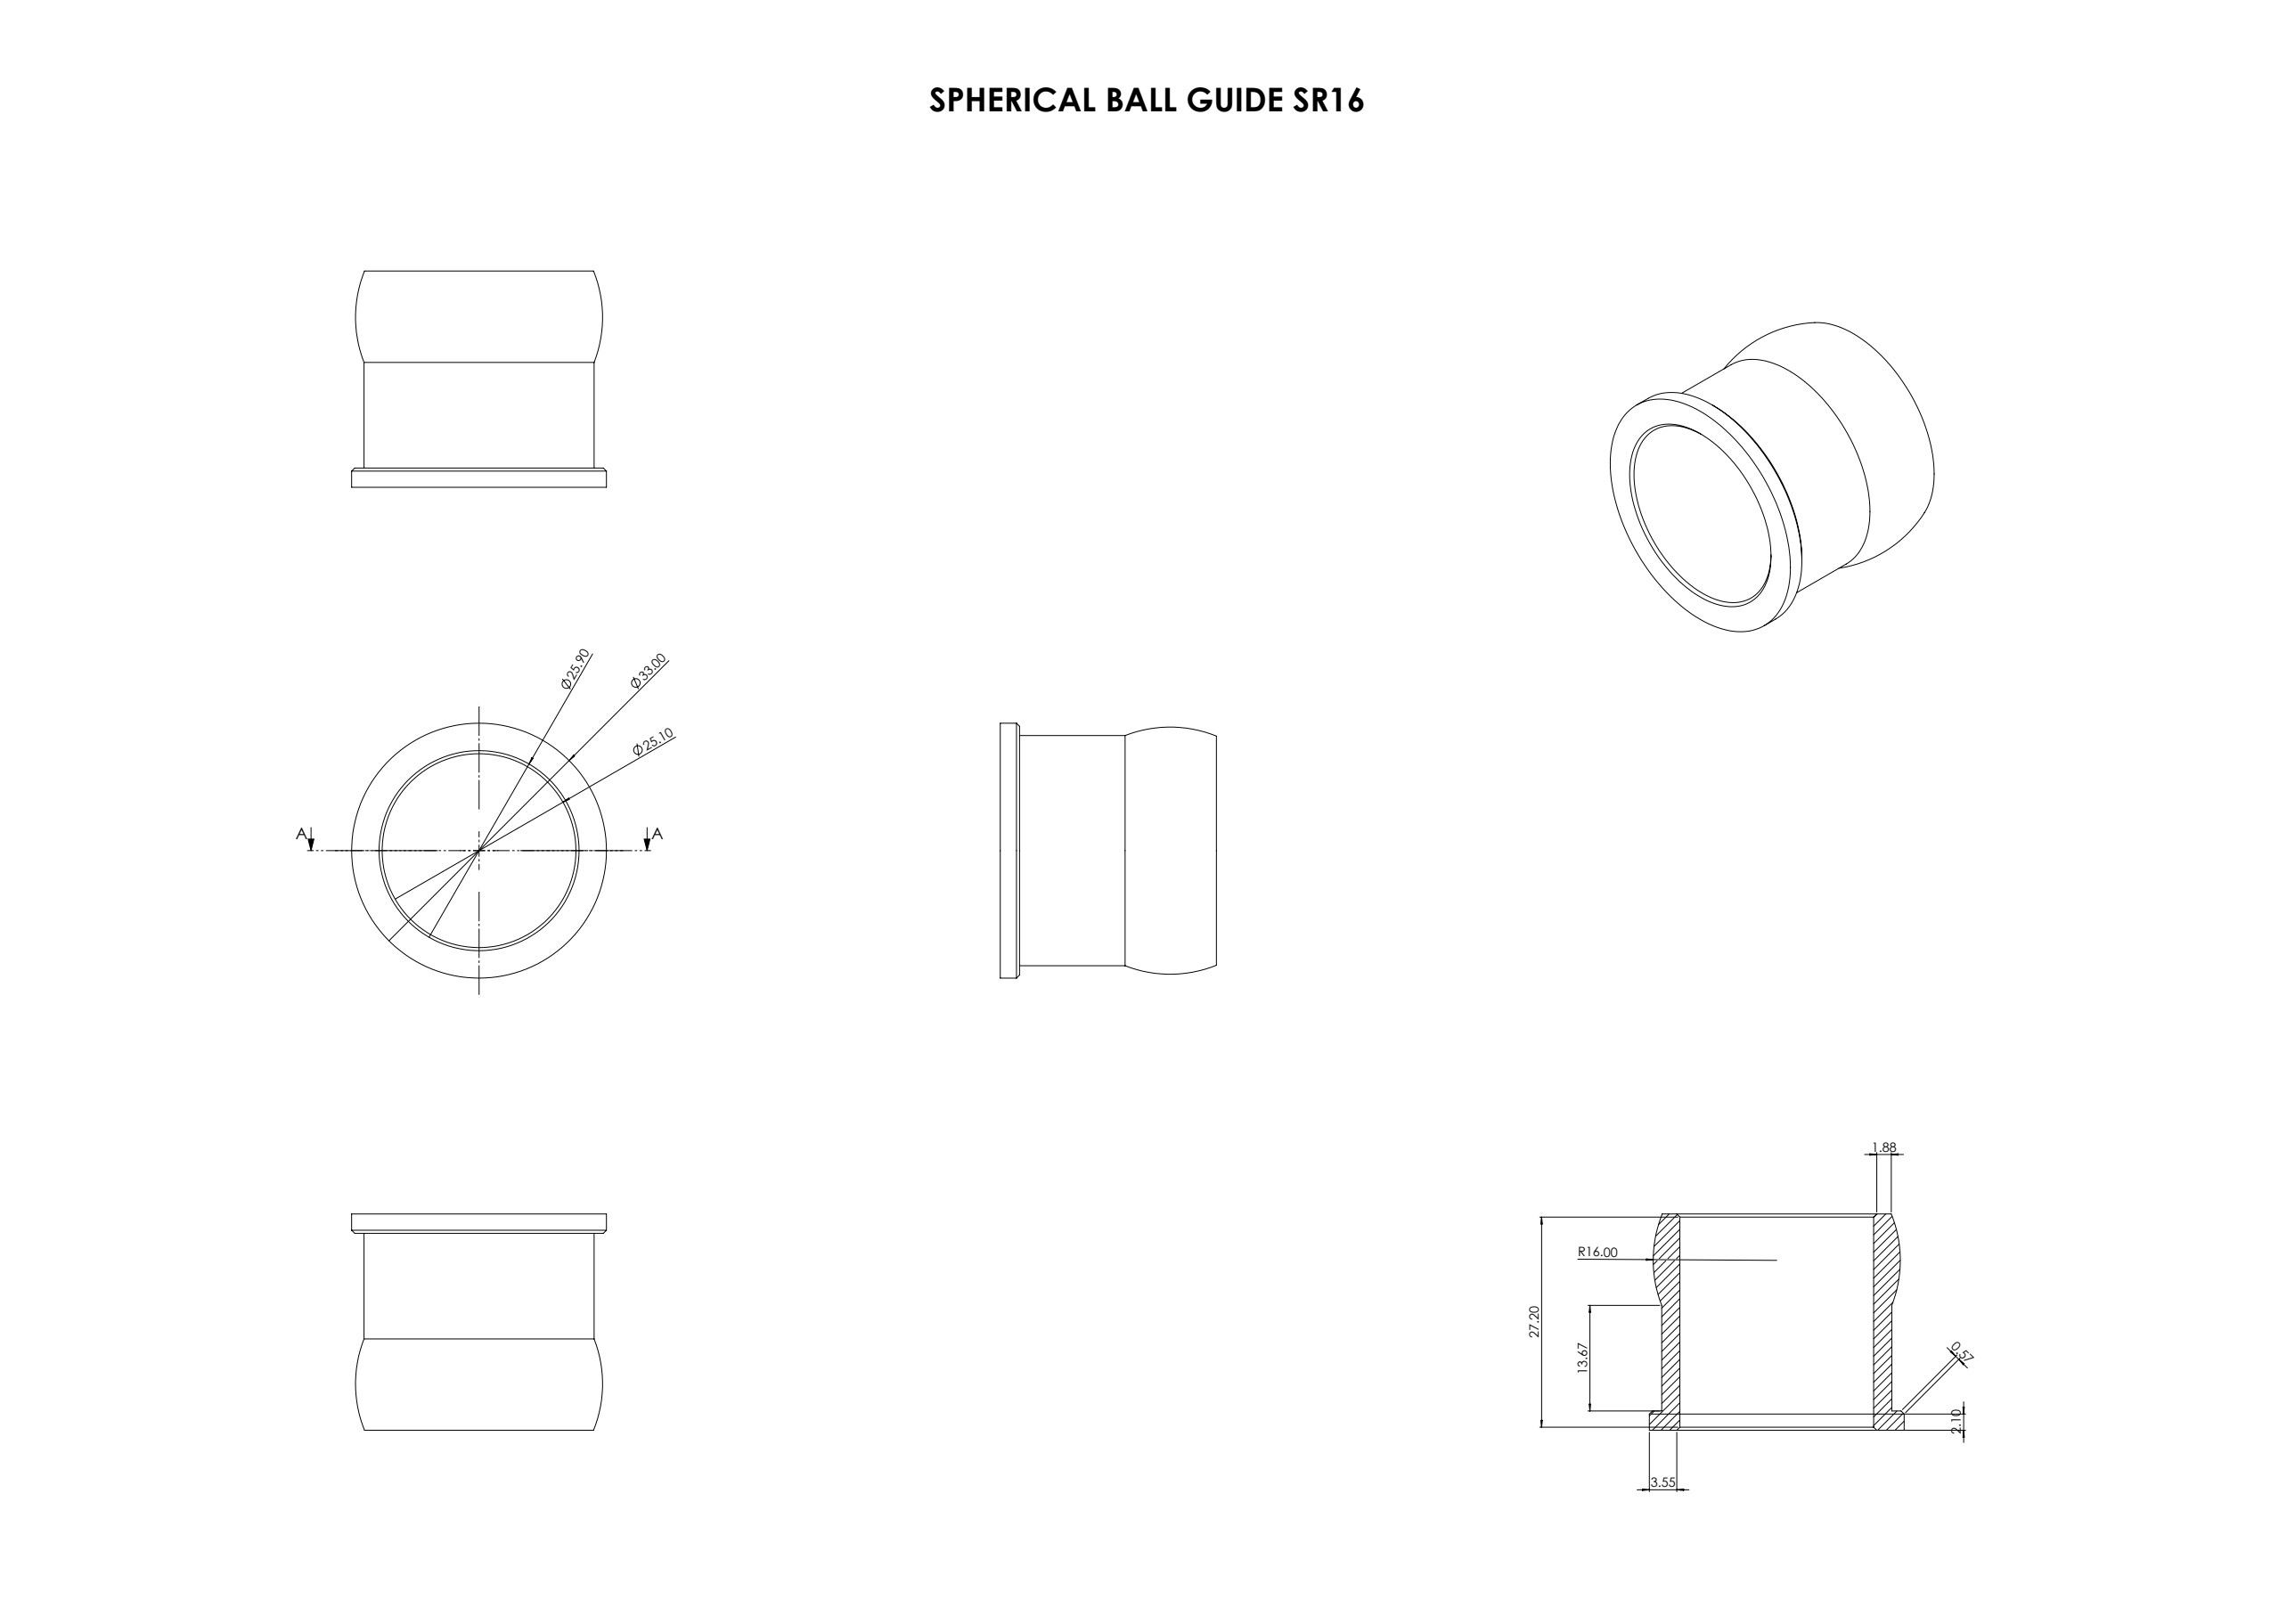
ISO-10303-21;
HEADER;
/* Generated by software containing ST-Developer
 * from STEP Tools, Inc. (www.steptools.com) 
 */

FILE_DESCRIPTION(
/* description */ (''),
/* implementation_level */ '2;1');

FILE_NAME(
/* name */ '09_Spherical_Ball_Guide_SR16.step',
/* time_stamp */ '2026-10-23T00:52:27+05:00',
/* author */ (''),
/* organization */ (''),
/* preprocessor_version */ 'ST-DEVELOPER v20.2',
/* originating_system */ 'Autodesk Translation Framework v15.15.0.0',
/* authorisation */ '');

FILE_SCHEMA (('AUTOMOTIVE_DESIGN { 1 0 10303 214 3 1 1 }'));
ENDSEC;

DATA;
#10=MECHANICAL_DESIGN_GEOMETRIC_PRESENTATION_REPRESENTATION('',(#1549),#59204);
#1509=SHAPE_REPRESENTATION_RELATIONSHIP('SRR','None',#59298,#1529);
#1529=ADVANCED_BREP_SHAPE_REPRESENTATION('',(#1576),#59185);
#1549=STYLED_ITEM('',(#59600),#1576);
#1576=MANIFOLD_SOLID_BREP('Ball guide',#22805);
#1596=SPHERICAL_SURFACE('',#23143,1.6);
#1619=FACE_BOUND('',#4029,.T.);
#1620=FACE_BOUND('',#4033,.T.);
#1621=FACE_BOUND('',#4038,.T.);
#1812=PLANE('',#23127);
#1813=PLANE('',#23133);
#1814=PLANE('',#23141);
#2419=CYLINDRICAL_SURFACE('',#23124,1.49);
#2420=CYLINDRICAL_SURFACE('',#23131,1.65);
#2421=CYLINDRICAL_SURFACE('',#23137,1.255);
#2702=FACE_OUTER_BOUND('',#4027,.T.);
#2703=FACE_OUTER_BOUND('',#4028,.T.);
#2704=FACE_OUTER_BOUND('',#4030,.T.);
#2705=FACE_OUTER_BOUND('',#4031,.T.);
#2706=FACE_OUTER_BOUND('',#4032,.T.);
#2707=FACE_OUTER_BOUND('',#4034,.T.);
#2708=FACE_OUTER_BOUND('',#4035,.T.);
#2709=FACE_OUTER_BOUND('',#4036,.T.);
#2710=FACE_OUTER_BOUND('',#4037,.T.);
#2711=FACE_OUTER_BOUND('',#4039,.T.);
#4027=EDGE_LOOP('',(#14808,#14809,#14810,#14811));
#4028=EDGE_LOOP('',(#14812));
#4029=EDGE_LOOP('',(#14813));
#4030=EDGE_LOOP('',(#14814,#14815,#14816,#14817));
#4031=EDGE_LOOP('',(#14818,#14819,#14820,#14821));
#4032=EDGE_LOOP('',(#14822));
#4033=EDGE_LOOP('',(#14823));
#4034=EDGE_LOOP('',(#14824,#14825,#14826,#14827));
#4035=EDGE_LOOP('',(#14828,#14829,#14830,#14831));
#4036=EDGE_LOOP('',(#14832,#14833,#14834,#14835));
#4037=EDGE_LOOP('',(#14836));
#4038=EDGE_LOOP('',(#14837));
#4039=EDGE_LOOP('',(#14838,#14839,#14840,#14841));
#5520=LINE('',#30846,#6953);
#5521=LINE('',#30854,#6954);
#5522=LINE('',#30858,#6955);
#5523=LINE('',#30864,#6956);
#5524=LINE('',#30868,#6957);
#5525=LINE('',#30872,#6958);
#6953=VECTOR('',#25308,1.49);
#6954=VECTOR('',#25319,1.63);
#6955=VECTOR('',#25324,1.65);
#6956=VECTOR('',#25331,1.275);
#6957=VECTOR('',#25336,1.255);
#6958=VECTOR('',#25341,1.275);
#8399=CIRCLE('',#23125,1.49);
#8400=CIRCLE('',#23126,1.49);
#8401=CIRCLE('',#23128,1.61);
#8402=CIRCLE('',#23130,1.65);
#8403=CIRCLE('',#23132,1.65);
#8404=CIRCLE('',#23134,1.295);
#8405=CIRCLE('',#23136,1.255);
#8406=CIRCLE('',#23138,1.255);
#8407=CIRCLE('',#23140,1.295);
#8408=CIRCLE('',#23142,1.48323969741913);
#8409=CIRCLE('',#23144,1.6);
#9234=VERTEX_POINT('',#30843);
#9235=VERTEX_POINT('',#30845);
#9236=VERTEX_POINT('',#30849);
#9237=VERTEX_POINT('',#30852);
#9238=VERTEX_POINT('',#30856);
#9239=VERTEX_POINT('',#30860);
#9240=VERTEX_POINT('',#30863);
#9241=VERTEX_POINT('',#30867);
#9242=VERTEX_POINT('',#30871);
#9243=VERTEX_POINT('',#30875);
#11408=EDGE_CURVE('',#9234,#9234,#8399,.T.);
#11409=EDGE_CURVE('',#9234,#9235,#5520,.T.);
#11410=EDGE_CURVE('',#9235,#9235,#8400,.T.);
#11411=EDGE_CURVE('',#9236,#9236,#8401,.T.);
#11412=EDGE_CURVE('',#9237,#9237,#8402,.T.);
#11413=EDGE_CURVE('',#9237,#9236,#5521,.T.);
#11414=EDGE_CURVE('',#9238,#9238,#8403,.T.);
#11415=EDGE_CURVE('',#9238,#9237,#5522,.T.);
#11416=EDGE_CURVE('',#9239,#9239,#8404,.T.);
#11417=EDGE_CURVE('',#9239,#9240,#5523,.T.);
#11418=EDGE_CURVE('',#9240,#9240,#8405,.T.);
#11419=EDGE_CURVE('',#9240,#9241,#5524,.T.);
#11420=EDGE_CURVE('',#9241,#9241,#8406,.T.);
#11421=EDGE_CURVE('',#9241,#9242,#5525,.T.);
#11422=EDGE_CURVE('',#9242,#9242,#8407,.T.);
#11423=EDGE_CURVE('',#9243,#9243,#8408,.T.);
#11424=EDGE_CURVE('',#9235,#9243,#8409,.T.);
#14808=ORIENTED_EDGE('',*,*,#11408,.F.);
#14809=ORIENTED_EDGE('',*,*,#11409,.T.);
#14810=ORIENTED_EDGE('',*,*,#11410,.T.);
#14811=ORIENTED_EDGE('',*,*,#11409,.F.);
#14812=ORIENTED_EDGE('',*,*,#11411,.F.);
#14813=ORIENTED_EDGE('',*,*,#11408,.T.);
#14814=ORIENTED_EDGE('',*,*,#11412,.F.);
#14815=ORIENTED_EDGE('',*,*,#11413,.T.);
#14816=ORIENTED_EDGE('',*,*,#11411,.T.);
#14817=ORIENTED_EDGE('',*,*,#11413,.F.);
#14818=ORIENTED_EDGE('',*,*,#11414,.F.);
#14819=ORIENTED_EDGE('',*,*,#11415,.T.);
#14820=ORIENTED_EDGE('',*,*,#11412,.T.);
#14821=ORIENTED_EDGE('',*,*,#11415,.F.);
#14822=ORIENTED_EDGE('',*,*,#11414,.T.);
#14823=ORIENTED_EDGE('',*,*,#11416,.F.);
#14824=ORIENTED_EDGE('',*,*,#11416,.T.);
#14825=ORIENTED_EDGE('',*,*,#11417,.T.);
#14826=ORIENTED_EDGE('',*,*,#11418,.F.);
#14827=ORIENTED_EDGE('',*,*,#11417,.F.);
#14828=ORIENTED_EDGE('',*,*,#11418,.T.);
#14829=ORIENTED_EDGE('',*,*,#11419,.T.);
#14830=ORIENTED_EDGE('',*,*,#11420,.F.);
#14831=ORIENTED_EDGE('',*,*,#11419,.F.);
#14832=ORIENTED_EDGE('',*,*,#11420,.T.);
#14833=ORIENTED_EDGE('',*,*,#11421,.T.);
#14834=ORIENTED_EDGE('',*,*,#11422,.F.);
#14835=ORIENTED_EDGE('',*,*,#11421,.F.);
#14836=ORIENTED_EDGE('',*,*,#11423,.F.);
#14837=ORIENTED_EDGE('',*,*,#11422,.T.);
#14838=ORIENTED_EDGE('',*,*,#11410,.F.);
#14839=ORIENTED_EDGE('',*,*,#11424,.T.);
#14840=ORIENTED_EDGE('',*,*,#11423,.T.);
#14841=ORIENTED_EDGE('',*,*,#11424,.F.);
#21336=CONICAL_SURFACE('',#23129,1.63,0.785398163397446);
#21337=CONICAL_SURFACE('',#23135,1.275,0.785398163397448);
#21338=CONICAL_SURFACE('',#23139,1.275,0.785398163397437);
#21532=ADVANCED_FACE('',(#2702),#2419,.T.);
#21533=ADVANCED_FACE('',(#2703,#1619),#1812,.T.);
#21534=ADVANCED_FACE('',(#2704),#21336,.T.);
#21535=ADVANCED_FACE('',(#2705),#2420,.T.);
#21536=ADVANCED_FACE('',(#2706,#1620),#1813,.T.);
#21537=ADVANCED_FACE('',(#2707),#21337,.F.);
#21538=ADVANCED_FACE('',(#2708),#2421,.F.);
#21539=ADVANCED_FACE('',(#2709),#21338,.F.);
#21540=ADVANCED_FACE('',(#2710,#1621),#1814,.T.);
#21541=ADVANCED_FACE('',(#2711),#1596,.T.);
#22805=CLOSED_SHELL('',(#21532,#21533,#21534,#21535,#21536,#21537,#21538,
#21539,#21540,#21541));
#23123=AXIS2_PLACEMENT_3D('',#30841,#25302,#25303);
#23124=AXIS2_PLACEMENT_3D('',#30842,#25304,#25305);
#23125=AXIS2_PLACEMENT_3D('',#30844,#25306,#25307);
#23126=AXIS2_PLACEMENT_3D('',#30847,#25309,#25310);
#23127=AXIS2_PLACEMENT_3D('',#30848,#25311,#25312);
#23128=AXIS2_PLACEMENT_3D('',#30850,#25313,#25314);
#23129=AXIS2_PLACEMENT_3D('',#30851,#25315,#25316);
#23130=AXIS2_PLACEMENT_3D('',#30853,#25317,#25318);
#23131=AXIS2_PLACEMENT_3D('',#30855,#25320,#25321);
#23132=AXIS2_PLACEMENT_3D('',#30857,#25322,#25323);
#23133=AXIS2_PLACEMENT_3D('',#30859,#25325,#25326);
#23134=AXIS2_PLACEMENT_3D('',#30861,#25327,#25328);
#23135=AXIS2_PLACEMENT_3D('',#30862,#25329,#25330);
#23136=AXIS2_PLACEMENT_3D('',#30865,#25332,#25333);
#23137=AXIS2_PLACEMENT_3D('',#30866,#25334,#25335);
#23138=AXIS2_PLACEMENT_3D('',#30869,#25337,#25338);
#23139=AXIS2_PLACEMENT_3D('',#30870,#25339,#25340);
#23140=AXIS2_PLACEMENT_3D('',#30873,#25342,#25343);
#23141=AXIS2_PLACEMENT_3D('',#30874,#25344,#25345);
#23142=AXIS2_PLACEMENT_3D('',#30876,#25346,#25347);
#23143=AXIS2_PLACEMENT_3D('',#30877,#25348,#25349);
#23144=AXIS2_PLACEMENT_3D('',#30878,#25350,#25351);
#25302=DIRECTION('axis',(0.,0.,1.));
#25303=DIRECTION('refdir',(1.,0.,0.));
#25304=DIRECTION('center_axis',(0.,0.,1.));
#25305=DIRECTION('ref_axis',(1.,0.,0.));
#25306=DIRECTION('center_axis',(0.,0.,1.));
#25307=DIRECTION('ref_axis',(1.,0.,0.));
#25308=DIRECTION('',(0.,0.,-1.));
#25309=DIRECTION('center_axis',(0.,0.,1.));
#25310=DIRECTION('ref_axis',(1.,0.,0.));
#25311=DIRECTION('center_axis',(0.,0.,-1.));
#25312=DIRECTION('ref_axis',(-1.,0.,0.));
#25313=DIRECTION('center_axis',(0.,0.,1.));
#25314=DIRECTION('ref_axis',(1.,0.,0.));
#25315=DIRECTION('center_axis',(0.,0.,1.));
#25316=DIRECTION('ref_axis',(1.,0.,0.));
#25317=DIRECTION('center_axis',(0.,0.,1.));
#25318=DIRECTION('ref_axis',(1.,0.,0.));
#25319=DIRECTION('',(0.707106781186545,8.65956056235491E-17,-0.707106781186549));
#25320=DIRECTION('center_axis',(0.,0.,1.));
#25321=DIRECTION('ref_axis',(1.,0.,0.));
#25322=DIRECTION('center_axis',(0.,0.,1.));
#25323=DIRECTION('ref_axis',(1.,0.,0.));
#25324=DIRECTION('',(0.,0.,-1.));
#25325=DIRECTION('center_axis',(0.,0.,1.));
#25326=DIRECTION('ref_axis',(1.,0.,0.));
#25327=DIRECTION('center_axis',(0.,0.,1.));
#25328=DIRECTION('ref_axis',(1.,0.,0.));
#25329=DIRECTION('center_axis',(0.,0.,1.));
#25330=DIRECTION('ref_axis',(1.,0.,0.));
#25331=DIRECTION('',(0.707106781186548,8.65956056235493E-17,-0.707106781186548));
#25332=DIRECTION('center_axis',(0.,0.,1.));
#25333=DIRECTION('ref_axis',(1.,0.,0.));
#25334=DIRECTION('center_axis',(0.,0.,1.));
#25335=DIRECTION('ref_axis',(1.,0.,0.));
#25336=DIRECTION('',(0.,0.,-1.));
#25337=DIRECTION('center_axis',(0.,0.,1.));
#25338=DIRECTION('ref_axis',(1.,0.,0.));
#25339=DIRECTION('center_axis',(0.,0.,-1.));
#25340=DIRECTION('ref_axis',(1.,0.,0.));
#25341=DIRECTION('',(-0.70710678118654,-8.65956056235484E-17,-0.707106781186555));
#25342=DIRECTION('center_axis',(0.,0.,1.));
#25343=DIRECTION('ref_axis',(1.,0.,0.));
#25344=DIRECTION('center_axis',(0.,0.,-1.));
#25345=DIRECTION('ref_axis',(-1.,0.,0.));
#25346=DIRECTION('center_axis',(0.,0.,1.));
#25347=DIRECTION('ref_axis',(1.,0.,0.));
#25348=DIRECTION('center_axis',(6.12323399573677E-17,0.,1.));
#25349=DIRECTION('ref_axis',(1.,0.,0.));
#25350=DIRECTION('center_axis',(1.22464679914735E-16,-1.,0.));
#25351=DIRECTION('ref_axis',(-1.,-1.22464679914735E-16,0.));
#30841=CARTESIAN_POINT('',(0.,0.,0.));
#30842=CARTESIAN_POINT('Origin',(0.,0.,-5.38349528305703));
#30843=CARTESIAN_POINT('',(-1.49,-1.82472373072956E-16,-4.7));
#30844=CARTESIAN_POINT('Origin',(0.,0.,-4.7));
#30845=CARTESIAN_POINT('',(-1.49,-1.82472373072956E-16,-6.06699056611406));
#30846=CARTESIAN_POINT('',(-1.49,-1.82472373072956E-16,-5.38349528305703));
#30847=CARTESIAN_POINT('Origin',(0.,0.,-6.06699056611406));
#30848=CARTESIAN_POINT('Origin',(1.61,0.,-4.7));
#30849=CARTESIAN_POINT('',(-1.61,-1.97168134662724E-16,-4.7));
#30850=CARTESIAN_POINT('Origin',(0.,0.,-4.7));
#30851=CARTESIAN_POINT('Origin',(0.,0.,-4.68));
#30852=CARTESIAN_POINT('',(-1.65,-2.02066721859313E-16,-4.66));
#30853=CARTESIAN_POINT('Origin',(0.,0.,-4.66));
#30854=CARTESIAN_POINT('',(-1.63,-1.99617428261019E-16,-4.68));
#30855=CARTESIAN_POINT('Origin',(0.,0.,-4.555));
#30856=CARTESIAN_POINT('',(-1.65,-2.02066721859313E-16,-4.45));
#30857=CARTESIAN_POINT('Origin',(0.,0.,-4.45));
#30858=CARTESIAN_POINT('',(-1.65,-2.02066721859313E-16,-4.555));
#30859=CARTESIAN_POINT('Origin',(1.295,0.,-4.45));
#30860=CARTESIAN_POINT('',(-1.295,-1.58591760489582E-16,-4.45));
#30861=CARTESIAN_POINT('Origin',(0.,0.,-4.45));
#30862=CARTESIAN_POINT('Origin',(0.,0.,-4.47));
#30863=CARTESIAN_POINT('',(-1.255,-1.53693173292993E-16,-4.49));
#30864=CARTESIAN_POINT('',(-1.275,-1.56142466891288E-16,-4.47));
#30865=CARTESIAN_POINT('Origin',(0.,0.,-4.49));
#30866=CARTESIAN_POINT('Origin',(0.,0.,-5.85));
#30867=CARTESIAN_POINT('',(-1.255,-1.53693173292993E-16,-7.21));
#30868=CARTESIAN_POINT('',(-1.255,-1.53693173292993E-16,-5.85));
#30869=CARTESIAN_POINT('Origin',(0.,0.,-7.21));
#30870=CARTESIAN_POINT('Origin',(0.,0.,-7.23));
#30871=CARTESIAN_POINT('',(-1.295,-1.58591760489582E-16,-7.25));
#30872=CARTESIAN_POINT('',(-1.275,-1.56142466891288E-16,-7.23));
#30873=CARTESIAN_POINT('Origin',(0.,0.,-7.25));
#30874=CARTESIAN_POINT('Origin',(1.48323969741913,0.,-7.25));
#30875=CARTESIAN_POINT('',(-1.48323969741913,-1.81644474781263E-16,-7.25));
#30876=CARTESIAN_POINT('Origin',(0.,0.,-7.25));
#30877=CARTESIAN_POINT('Origin',(2.22044604925031E-16,0.,-6.65));
#30878=CARTESIAN_POINT('Origin',(2.22044604925031E-16,0.,-6.65));
#59163=UNCERTAINTY_MEASURE_WITH_UNIT(LENGTH_MEASURE(0.001),#59205,
'DISTANCE_ACCURACY_VALUE',
'Maximum model space distance between geometric entities at asserted c
onnectivities');
#59182=UNCERTAINTY_MEASURE_WITH_UNIT(LENGTH_MEASURE(0.001),#59205,
'DISTANCE_ACCURACY_VALUE',
'Maximum model space distance between geometric entities at asserted c
onnectivities');
#59185=(
GEOMETRIC_REPRESENTATION_CONTEXT(3)
GLOBAL_UNCERTAINTY_ASSIGNED_CONTEXT((#59163))
GLOBAL_UNIT_ASSIGNED_CONTEXT((#59205,#59207,#59208))
REPRESENTATION_CONTEXT('','3D')
);
#59204=(
GEOMETRIC_REPRESENTATION_CONTEXT(3)
GLOBAL_UNCERTAINTY_ASSIGNED_CONTEXT((#59182))
GLOBAL_UNIT_ASSIGNED_CONTEXT((#59205,#59207,#59208))
REPRESENTATION_CONTEXT('','3D')
);
#59205=(
LENGTH_UNIT()
NAMED_UNIT(*)
SI_UNIT(.CENTI.,.METRE.)
);
#59207=(
NAMED_UNIT(*)
PLANE_ANGLE_UNIT()
SI_UNIT($,.RADIAN.)
);
#59208=(
NAMED_UNIT(*)
SI_UNIT($,.STERADIAN.)
SOLID_ANGLE_UNIT()
);
#59211=SHAPE_DEFINITION_REPRESENTATION(#59232,#59298);
#59232=PRODUCT_DEFINITION_SHAPE('',$,#59320);
#59298=SHAPE_REPRESENTATION('',(#23123),#59185);
#59317=PRODUCT_DEFINITION_CONTEXT('part definition',#59382,'design');
#59320=PRODUCT_DEFINITION('2026-10-23-00-47-19-123',
'09_Spherical_Ball_Guide_SR16',#59341,#59317);
#59341=PRODUCT_DEFINITION_FORMATION('',$,#59386);
#59382=APPLICATION_CONTEXT(
'Core Data for Automotive Mechanical Design Process');
#59383=PRODUCT_CONTEXT('part definition',#59382,'mechanical');
#59386=PRODUCT('2026-10-23-00-47-19-123','09_Spherical_Ball_Guide_SR16',
$,(#59383));
#59594=COLOUR_RGB('Off White',0.89,0.88,0.83);
#59595=FILL_AREA_STYLE_COLOUR('',#59594);
#59596=FILL_AREA_STYLE('',(#59595));
#59597=SURFACE_STYLE_FILL_AREA(#59596);
#59598=SURFACE_SIDE_STYLE('',(#59597));
#59599=SURFACE_STYLE_USAGE(.BOTH.,#59598);
#59600=PRESENTATION_STYLE_ASSIGNMENT((#59599));
ENDSEC;
END-ISO-10303-21;
